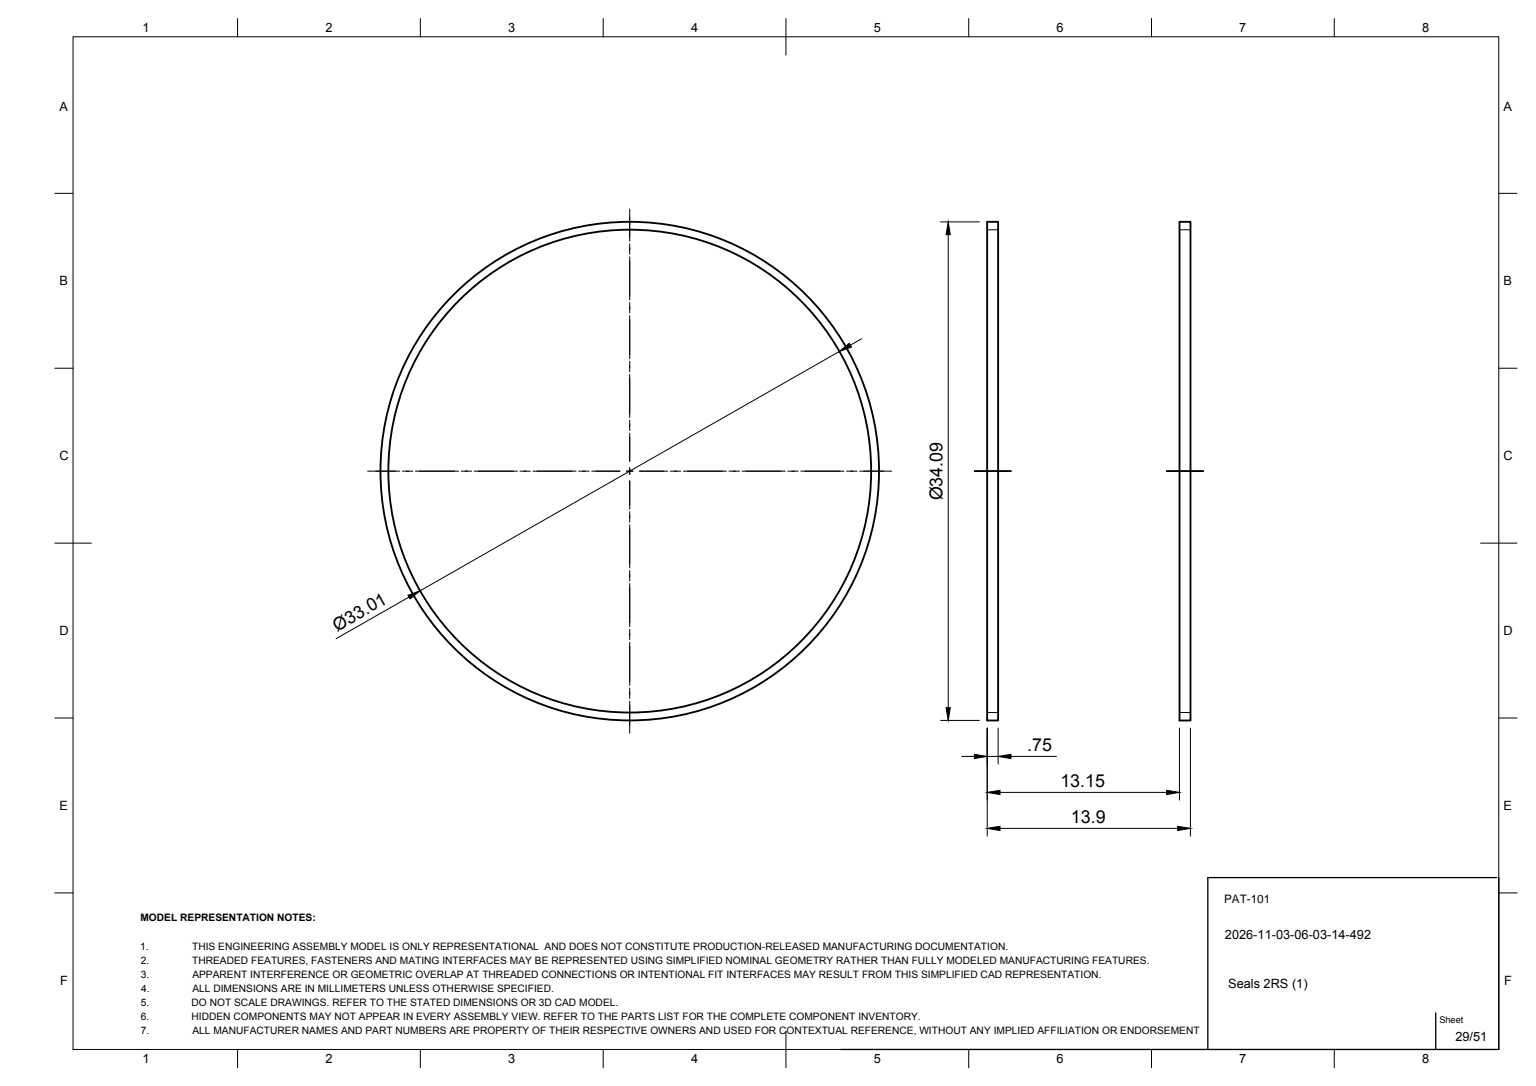
ISO-10303-21;
HEADER;
/* Generated by software containing ST-Developer
 * from STEP Tools, Inc. (www.steptools.com) 
 */

FILE_DESCRIPTION(
/* description */ ('Spur gear reduction stage 2-1 on bearing plates'),
/* implementation_level */ '2;1');

FILE_NAME(
/* name */ 'Seals 2RS (1).step',
/* time_stamp */ '2026-10-28T03:22:07-07:00',
/* author */ (''),
/* organization */ (''),
/* preprocessor_version */ 'ST-DEVELOPER v20.2',
/* originating_system */ 'Autodesk Translation Framework v15.17.0.0',
/* authorisation */ '');

FILE_SCHEMA (('AUTOMOTIVE_DESIGN { 1 0 10303 214 3 1 1 }'));
ENDSEC;

DATA;
#10=MECHANICAL_DESIGN_GEOMETRIC_PRESENTATION_REPRESENTATION('',(#983,#984),#53909);
#883=SHAPE_REPRESENTATION_RELATIONSHIP('SRR','None',#54112,#926);
#926=ADVANCED_BREP_SHAPE_REPRESENTATION('',(#1039,#1040),#53886);
#983=STYLED_ITEM('',(#54397),#1039);
#984=STYLED_ITEM('',(#54397),#1040);
#1039=MANIFOLD_SOLID_BREP('Body1',#11309);
#1040=MANIFOLD_SOLID_BREP('Body2',#11310);
#1192=FACE_BOUND('',#2539,.T.);
#1193=FACE_BOUND('',#2542,.T.);
#1194=FACE_BOUND('',#2545,.T.);
#1195=FACE_BOUND('',#2548,.T.);
#1343=PLANE('',#12394);
#1344=PLANE('',#12399);
#1345=PLANE('',#12402);
#1346=PLANE('',#12407);
#1758=FACE_OUTER_BOUND('',#2538,.T.);
#1759=FACE_OUTER_BOUND('',#2540,.T.);
#1760=FACE_OUTER_BOUND('',#2541,.T.);
#1761=FACE_OUTER_BOUND('',#2543,.T.);
#1762=FACE_OUTER_BOUND('',#2544,.T.);
#1763=FACE_OUTER_BOUND('',#2546,.T.);
#1764=FACE_OUTER_BOUND('',#2547,.T.);
#1765=FACE_OUTER_BOUND('',#2549,.T.);
#2538=EDGE_LOOP('',(#8394));
#2539=EDGE_LOOP('',(#8395));
#2540=EDGE_LOOP('',(#8396,#8397,#8398,#8399));
#2541=EDGE_LOOP('',(#8400));
#2542=EDGE_LOOP('',(#8401));
#2543=EDGE_LOOP('',(#8402,#8403,#8404,#8405));
#2544=EDGE_LOOP('',(#8406));
#2545=EDGE_LOOP('',(#8407));
#2546=EDGE_LOOP('',(#8408,#8409,#8410,#8411));
#2547=EDGE_LOOP('',(#8412));
#2548=EDGE_LOOP('',(#8413));
#2549=EDGE_LOOP('',(#8414,#8415,#8416,#8417));
#3165=LINE('',#17785,#3806);
#3166=LINE('',#17790,#3807);
#3167=LINE('',#17799,#3808);
#3168=LINE('',#17804,#3809);
#3806=VECTOR('',#14356,1.70469);
#3807=VECTOR('',#14363,1.65031);
#3808=VECTOR('',#14374,1.70469);
#3809=VECTOR('',#14381,1.65031);
#4560=CIRCLE('',#12395,1.70469);
#4561=CIRCLE('',#12396,1.65031);
#4562=CIRCLE('',#12398,1.70469);
#4563=CIRCLE('',#12400,1.65031);
#4564=CIRCLE('',#12403,1.70469);
#4565=CIRCLE('',#12404,1.65031);
#4566=CIRCLE('',#12406,1.70469);
#4567=CIRCLE('',#12408,1.65031);
#5146=VERTEX_POINT('',#17778);
#5147=VERTEX_POINT('',#17780);
#5148=VERTEX_POINT('',#17783);
#5149=VERTEX_POINT('',#17787);
#5150=VERTEX_POINT('',#17792);
#5151=VERTEX_POINT('',#17794);
#5152=VERTEX_POINT('',#17797);
#5153=VERTEX_POINT('',#17801);
#6339=EDGE_CURVE('',#5146,#5146,#4560,.T.);
#6340=EDGE_CURVE('',#5147,#5147,#4561,.T.);
#6341=EDGE_CURVE('',#5148,#5148,#4562,.T.);
#6342=EDGE_CURVE('',#5148,#5146,#3165,.T.);
#6343=EDGE_CURVE('',#5149,#5149,#4563,.T.);
#6344=EDGE_CURVE('',#5149,#5147,#3166,.T.);
#6345=EDGE_CURVE('',#5150,#5150,#4564,.T.);
#6346=EDGE_CURVE('',#5151,#5151,#4565,.T.);
#6347=EDGE_CURVE('',#5152,#5152,#4566,.T.);
#6348=EDGE_CURVE('',#5152,#5150,#3167,.T.);
#6349=EDGE_CURVE('',#5153,#5153,#4567,.T.);
#6350=EDGE_CURVE('',#5153,#5151,#3168,.T.);
#8394=ORIENTED_EDGE('',*,*,#6339,.F.);
#8395=ORIENTED_EDGE('',*,*,#6340,.T.);
#8396=ORIENTED_EDGE('',*,*,#6341,.F.);
#8397=ORIENTED_EDGE('',*,*,#6342,.T.);
#8398=ORIENTED_EDGE('',*,*,#6339,.T.);
#8399=ORIENTED_EDGE('',*,*,#6342,.F.);
#8400=ORIENTED_EDGE('',*,*,#6341,.T.);
#8401=ORIENTED_EDGE('',*,*,#6343,.F.);
#8402=ORIENTED_EDGE('',*,*,#6343,.T.);
#8403=ORIENTED_EDGE('',*,*,#6344,.T.);
#8404=ORIENTED_EDGE('',*,*,#6340,.F.);
#8405=ORIENTED_EDGE('',*,*,#6344,.F.);
#8406=ORIENTED_EDGE('',*,*,#6345,.F.);
#8407=ORIENTED_EDGE('',*,*,#6346,.T.);
#8408=ORIENTED_EDGE('',*,*,#6347,.F.);
#8409=ORIENTED_EDGE('',*,*,#6348,.T.);
#8410=ORIENTED_EDGE('',*,*,#6345,.T.);
#8411=ORIENTED_EDGE('',*,*,#6348,.F.);
#8412=ORIENTED_EDGE('',*,*,#6347,.T.);
#8413=ORIENTED_EDGE('',*,*,#6349,.F.);
#8414=ORIENTED_EDGE('',*,*,#6349,.T.);
#8415=ORIENTED_EDGE('',*,*,#6350,.T.);
#8416=ORIENTED_EDGE('',*,*,#6346,.F.);
#8417=ORIENTED_EDGE('',*,*,#6350,.F.);
#10520=CYLINDRICAL_SURFACE('',#12397,1.70469);
#10521=CYLINDRICAL_SURFACE('',#12401,1.65031);
#10522=CYLINDRICAL_SURFACE('',#12405,1.70469);
#10523=CYLINDRICAL_SURFACE('',#12409,1.65031);
#10878=ADVANCED_FACE('',(#1758,#1192),#1343,.T.);
#10879=ADVANCED_FACE('',(#1759),#10520,.T.);
#10880=ADVANCED_FACE('',(#1760,#1193),#1344,.T.);
#10881=ADVANCED_FACE('',(#1761),#10521,.F.);
#10882=ADVANCED_FACE('',(#1762,#1194),#1345,.T.);
#10883=ADVANCED_FACE('',(#1763),#10522,.T.);
#10884=ADVANCED_FACE('',(#1764,#1195),#1346,.T.);
#10885=ADVANCED_FACE('',(#1765),#10523,.F.);
#11309=CLOSED_SHELL('',(#10878,#10879,#10880,#10881));
#11310=CLOSED_SHELL('',(#10882,#10883,#10884,#10885));
#12393=AXIS2_PLACEMENT_3D('',#17776,#14344,#14345);
#12394=AXIS2_PLACEMENT_3D('',#17777,#14346,#14347);
#12395=AXIS2_PLACEMENT_3D('',#17779,#14348,#14349);
#12396=AXIS2_PLACEMENT_3D('',#17781,#14350,#14351);
#12397=AXIS2_PLACEMENT_3D('',#17782,#14352,#14353);
#12398=AXIS2_PLACEMENT_3D('',#17784,#14354,#14355);
#12399=AXIS2_PLACEMENT_3D('',#17786,#14357,#14358);
#12400=AXIS2_PLACEMENT_3D('',#17788,#14359,#14360);
#12401=AXIS2_PLACEMENT_3D('',#17789,#14361,#14362);
#12402=AXIS2_PLACEMENT_3D('',#17791,#14364,#14365);
#12403=AXIS2_PLACEMENT_3D('',#17793,#14366,#14367);
#12404=AXIS2_PLACEMENT_3D('',#17795,#14368,#14369);
#12405=AXIS2_PLACEMENT_3D('',#17796,#14370,#14371);
#12406=AXIS2_PLACEMENT_3D('',#17798,#14372,#14373);
#12407=AXIS2_PLACEMENT_3D('',#17800,#14375,#14376);
#12408=AXIS2_PLACEMENT_3D('',#17802,#14377,#14378);
#12409=AXIS2_PLACEMENT_3D('',#17803,#14379,#14380);
#14344=DIRECTION('axis',(0.,0.,1.));
#14345=DIRECTION('refdir',(1.,0.,0.));
#14346=DIRECTION('center_axis',(0.,1.,0.));
#14347=DIRECTION('ref_axis',(0.,0.,1.));
#14348=DIRECTION('center_axis',(0.,-1.,0.));
#14349=DIRECTION('ref_axis',(1.,0.,0.));
#14350=DIRECTION('center_axis',(0.,-1.,0.));
#14351=DIRECTION('ref_axis',(1.,0.,0.));
#14352=DIRECTION('center_axis',(0.,-1.,0.));
#14353=DIRECTION('ref_axis',(1.,0.,0.));
#14354=DIRECTION('center_axis',(0.,-1.,0.));
#14355=DIRECTION('ref_axis',(1.,0.,0.));
#14356=DIRECTION('',(0.,1.,0.));
#14357=DIRECTION('center_axis',(0.,-1.,0.));
#14358=DIRECTION('ref_axis',(0.,0.,-1.));
#14359=DIRECTION('center_axis',(0.,-1.,0.));
#14360=DIRECTION('ref_axis',(1.,0.,0.));
#14361=DIRECTION('center_axis',(0.,-1.,0.));
#14362=DIRECTION('ref_axis',(1.,0.,0.));
#14363=DIRECTION('',(0.,1.,0.));
#14364=DIRECTION('center_axis',(0.,1.,0.));
#14365=DIRECTION('ref_axis',(0.,0.,1.));
#14366=DIRECTION('center_axis',(0.,-1.,0.));
#14367=DIRECTION('ref_axis',(1.,0.,0.));
#14368=DIRECTION('center_axis',(0.,-1.,0.));
#14369=DIRECTION('ref_axis',(1.,0.,0.));
#14370=DIRECTION('center_axis',(0.,-1.,0.));
#14371=DIRECTION('ref_axis',(1.,0.,0.));
#14372=DIRECTION('center_axis',(0.,-1.,0.));
#14373=DIRECTION('ref_axis',(1.,0.,0.));
#14374=DIRECTION('',(0.,1.,0.));
#14375=DIRECTION('center_axis',(0.,-1.,0.));
#14376=DIRECTION('ref_axis',(0.,0.,-1.));
#14377=DIRECTION('center_axis',(0.,-1.,0.));
#14378=DIRECTION('ref_axis',(1.,0.,0.));
#14379=DIRECTION('center_axis',(0.,-1.,0.));
#14380=DIRECTION('ref_axis',(1.,0.,0.));
#14381=DIRECTION('',(0.,1.,0.));
#17776=CARTESIAN_POINT('',(0.,0.,0.));
#17777=CARTESIAN_POINT('Origin',(1.70469,0.695,0.));
#17778=CARTESIAN_POINT('',(-1.70469,0.695,-2.0876431520385E-16));
#17779=CARTESIAN_POINT('Origin',(0.,0.695,0.));
#17780=CARTESIAN_POINT('',(-1.65031,0.695,-2.02104685910087E-16));
#17781=CARTESIAN_POINT('Origin',(0.,0.695,0.));
#17782=CARTESIAN_POINT('Origin',(0.,0.6575,0.));
#17783=CARTESIAN_POINT('',(-1.70469,0.62,-2.0876431520385E-16));
#17784=CARTESIAN_POINT('Origin',(0.,0.62,0.));
#17785=CARTESIAN_POINT('',(-1.70469,0.6575,-2.0876431520385E-16));
#17786=CARTESIAN_POINT('Origin',(1.65031,0.62,0.));
#17787=CARTESIAN_POINT('',(-1.65031,0.62,-2.02104685910087E-16));
#17788=CARTESIAN_POINT('Origin',(0.,0.62,0.));
#17789=CARTESIAN_POINT('Origin',(0.,0.6575,0.));
#17790=CARTESIAN_POINT('',(-1.65031,0.6575,-2.02104685910087E-16));
#17791=CARTESIAN_POINT('Origin',(1.70469,-0.62,0.));
#17792=CARTESIAN_POINT('',(-1.70469,-0.62,-2.0876431520385E-16));
#17793=CARTESIAN_POINT('Origin',(0.,-0.62,0.));
#17794=CARTESIAN_POINT('',(-1.65031,-0.62,-2.02104685910087E-16));
#17795=CARTESIAN_POINT('Origin',(0.,-0.62,0.));
#17796=CARTESIAN_POINT('Origin',(0.,-0.6575,0.));
#17797=CARTESIAN_POINT('',(-1.70469,-0.695,-2.0876431520385E-16));
#17798=CARTESIAN_POINT('Origin',(0.,-0.695,0.));
#17799=CARTESIAN_POINT('',(-1.70469,-0.6575,-2.0876431520385E-16));
#17800=CARTESIAN_POINT('Origin',(1.65031,-0.695,0.));
#17801=CARTESIAN_POINT('',(-1.65031,-0.695,-2.02104685910087E-16));
#17802=CARTESIAN_POINT('Origin',(0.,-0.695,0.));
#17803=CARTESIAN_POINT('Origin',(0.,-0.6575,0.));
#17804=CARTESIAN_POINT('',(-1.65031,-0.6575,-2.02104685910087E-16));
#53836=UNCERTAINTY_MEASURE_WITH_UNIT(LENGTH_MEASURE(0.001),#53910,
'DISTANCE_ACCURACY_VALUE',
'Maximum model space distance between geometric entities at asserted c
onnectivities');
#53859=UNCERTAINTY_MEASURE_WITH_UNIT(LENGTH_MEASURE(0.001),#53910,
'DISTANCE_ACCURACY_VALUE',
'Maximum model space distance between geometric entities at asserted c
onnectivities');
#53886=(
GEOMETRIC_REPRESENTATION_CONTEXT(3)
GLOBAL_UNCERTAINTY_ASSIGNED_CONTEXT((#53836))
GLOBAL_UNIT_ASSIGNED_CONTEXT((#53910,#53912,#53913))
REPRESENTATION_CONTEXT('','3D')
);
#53909=(
GEOMETRIC_REPRESENTATION_CONTEXT(3)
GLOBAL_UNCERTAINTY_ASSIGNED_CONTEXT((#53859))
GLOBAL_UNIT_ASSIGNED_CONTEXT((#53910,#53912,#53913))
REPRESENTATION_CONTEXT('','3D')
);
#53910=(
LENGTH_UNIT()
NAMED_UNIT(*)
SI_UNIT(.CENTI.,.METRE.)
);
#53912=(
NAMED_UNIT(*)
PLANE_ANGLE_UNIT()
SI_UNIT($,.RADIAN.)
);
#53913=(
NAMED_UNIT(*)
SI_UNIT($,.STERADIAN.)
SOLID_ANGLE_UNIT()
);
#53940=SHAPE_DEFINITION_REPRESENTATION(#53994,#54112);
#53994=PRODUCT_DEFINITION_SHAPE('',$,#54162);
#54112=SHAPE_REPRESENTATION('',(#12393),#53886);
#54135=PRODUCT_DEFINITION_CONTEXT('part definition',#54284,'design');
#54162=PRODUCT_DEFINITION('Seals 2RS (1)','Seals 2RS (1)',#54211,#54135);
#54211=PRODUCT_DEFINITION_FORMATION('',$,#54312);
#54284=APPLICATION_CONTEXT(
'Core Data for Automotive Mechanical Design Process');
#54285=PRODUCT_CONTEXT('part definition',#54284,'mechanical');
#54312=PRODUCT('Seals 2RS (1)','Seals 2RS (1)','Seals 2RS (1)',(#54285));
#54391=COLOUR_RGB('Grey',0.48,0.52,0.57);
#54392=FILL_AREA_STYLE_COLOUR('',#54391);
#54393=FILL_AREA_STYLE('',(#54392));
#54394=SURFACE_STYLE_FILL_AREA(#54393);
#54395=SURFACE_SIDE_STYLE('',(#54394));
#54396=SURFACE_STYLE_USAGE(.BOTH.,#54395);
#54397=PRESENTATION_STYLE_ASSIGNMENT((#54396));
ENDSEC;
END-ISO-10303-21;
